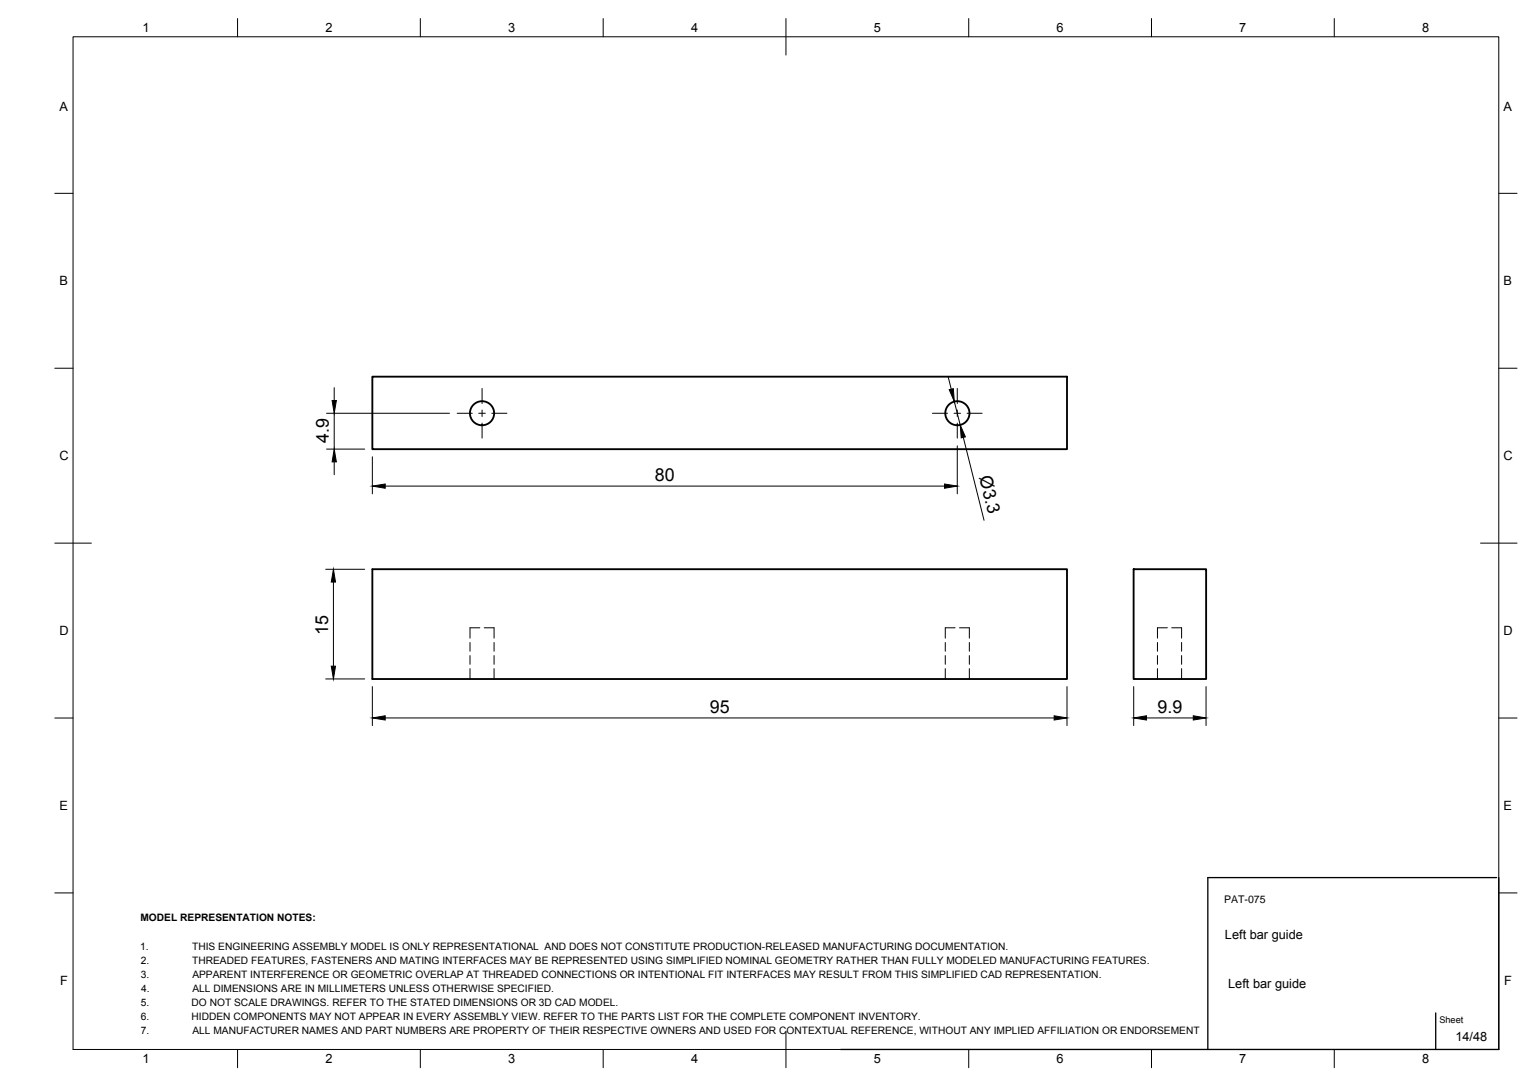
ISO-10303-21;
HEADER;
/* Generated by software containing ST-Developer
 * from STEP Tools, Inc. (www.steptools.com) 
 */

FILE_DESCRIPTION(
/* description */ ('Over-Centre Plunger Toggle Clamp on Slotted Fixture Frame'),
/* implementation_level */ '2;1');

FILE_NAME(
/* name */ 
'Left bar guide.step',
/* time_stamp */ '2026-10-28T03:23:24-07:00',
/* author */ (''),
/* organization */ (''),
/* preprocessor_version */ 'ST-DEVELOPER v20.2',
/* originating_system */ 'Autodesk Translation Framework v15.17.0.0',
/* authorisation */ '');

FILE_SCHEMA (('AUTOMOTIVE_DESIGN { 1 0 10303 214 3 1 1 }'));
ENDSEC;

DATA;
#10=MECHANICAL_DESIGN_GEOMETRIC_PRESENTATION_REPRESENTATION('',(#522),#15212);
#438=SHAPE_REPRESENTATION_RELATIONSHIP('SRR','None',#15412,#480);
#480=ADVANCED_BREP_SHAPE_REPRESENTATION('',(#573),#15174);
#522=STYLED_ITEM('',(#15712),#573);
#573=MANIFOLD_SOLID_BREP('Body1',#8254);
#708=FACE_BOUND('',#1802,.T.);
#709=FACE_BOUND('',#1803,.T.);
#846=PLANE('',#9018);
#847=PLANE('',#9022);
#848=PLANE('',#9023);
#849=PLANE('',#9024);
#850=PLANE('',#9025);
#851=PLANE('',#9026);
#852=PLANE('',#9027);
#853=PLANE('',#9028);
#1209=FACE_OUTER_BOUND('',#1792,.T.);
#1210=FACE_OUTER_BOUND('',#1793,.T.);
#1211=FACE_OUTER_BOUND('',#1794,.T.);
#1212=FACE_OUTER_BOUND('',#1795,.T.);
#1213=FACE_OUTER_BOUND('',#1796,.T.);
#1214=FACE_OUTER_BOUND('',#1797,.T.);
#1215=FACE_OUTER_BOUND('',#1798,.T.);
#1216=FACE_OUTER_BOUND('',#1799,.T.);
#1217=FACE_OUTER_BOUND('',#1800,.T.);
#1218=FACE_OUTER_BOUND('',#1801,.T.);
#1792=EDGE_LOOP('',(#6115,#6116,#6117,#6118));
#1793=EDGE_LOOP('',(#6119));
#1794=EDGE_LOOP('',(#6120,#6121,#6122,#6123));
#1795=EDGE_LOOP('',(#6124));
#1796=EDGE_LOOP('',(#6125,#6126,#6127,#6128));
#1797=EDGE_LOOP('',(#6129,#6130,#6131,#6132));
#1798=EDGE_LOOP('',(#6133,#6134,#6135,#6136));
#1799=EDGE_LOOP('',(#6137,#6138,#6139,#6140));
#1800=EDGE_LOOP('',(#6141,#6142,#6143,#6144));
#1801=EDGE_LOOP('',(#6145,#6146,#6147,#6148));
#1802=EDGE_LOOP('',(#6149));
#1803=EDGE_LOOP('',(#6150));
#2386=LINE('',#12959,#3016);
#2387=LINE('',#12966,#3017);
#2388=LINE('',#12972,#3018);
#2389=LINE('',#12974,#3019);
#2390=LINE('',#12976,#3020);
#2391=LINE('',#12977,#3021);
#2392=LINE('',#12980,#3022);
#2393=LINE('',#12982,#3023);
#2394=LINE('',#12983,#3024);
#2395=LINE('',#12986,#3025);
#2396=LINE('',#12988,#3026);
#2397=LINE('',#12989,#3027);
#2398=LINE('',#12991,#3028);
#2399=LINE('',#12992,#3029);
#3016=VECTOR('',#10417,0.165);
#3017=VECTOR('',#10426,0.165);
#3018=VECTOR('',#10433,1.);
#3019=VECTOR('',#10434,1.);
#3020=VECTOR('',#10435,1.);
#3021=VECTOR('',#10436,1.);
#3022=VECTOR('',#10439,1.);
#3023=VECTOR('',#10440,1.);
#3024=VECTOR('',#10441,1.);
#3025=VECTOR('',#10444,1.);
#3026=VECTOR('',#10445,1.);
#3027=VECTOR('',#10446,1.);
#3028=VECTOR('',#10449,1.);
#3029=VECTOR('',#10450,1.);
#3609=CIRCLE('',#9016,0.165);
#3610=CIRCLE('',#9017,0.165);
#3611=CIRCLE('',#9020,0.165);
#3612=CIRCLE('',#9021,0.165);
#4041=VERTEX_POINT('',#12956);
#4042=VERTEX_POINT('',#12958);
#4043=VERTEX_POINT('',#12963);
#4044=VERTEX_POINT('',#12965);
#4045=VERTEX_POINT('',#12970);
#4046=VERTEX_POINT('',#12971);
#4047=VERTEX_POINT('',#12973);
#4048=VERTEX_POINT('',#12975);
#4049=VERTEX_POINT('',#12979);
#4050=VERTEX_POINT('',#12981);
#4051=VERTEX_POINT('',#12985);
#4052=VERTEX_POINT('',#12987);
#4818=EDGE_CURVE('',#4041,#4041,#3609,.T.);
#4819=EDGE_CURVE('',#4041,#4042,#2386,.T.);
#4820=EDGE_CURVE('',#4042,#4042,#3610,.T.);
#4821=EDGE_CURVE('',#4043,#4043,#3611,.T.);
#4822=EDGE_CURVE('',#4043,#4044,#2387,.T.);
#4823=EDGE_CURVE('',#4044,#4044,#3612,.T.);
#4824=EDGE_CURVE('',#4045,#4046,#2388,.T.);
#4825=EDGE_CURVE('',#4046,#4047,#2389,.T.);
#4826=EDGE_CURVE('',#4048,#4047,#2390,.T.);
#4827=EDGE_CURVE('',#4045,#4048,#2391,.T.);
#4828=EDGE_CURVE('',#4049,#4045,#2392,.T.);
#4829=EDGE_CURVE('',#4050,#4048,#2393,.T.);
#4830=EDGE_CURVE('',#4049,#4050,#2394,.T.);
#4831=EDGE_CURVE('',#4051,#4049,#2395,.T.);
#4832=EDGE_CURVE('',#4052,#4050,#2396,.T.);
#4833=EDGE_CURVE('',#4051,#4052,#2397,.T.);
#4834=EDGE_CURVE('',#4046,#4051,#2398,.T.);
#4835=EDGE_CURVE('',#4047,#4052,#2399,.T.);
#6115=ORIENTED_EDGE('',*,*,#4818,.F.);
#6116=ORIENTED_EDGE('',*,*,#4819,.T.);
#6117=ORIENTED_EDGE('',*,*,#4820,.T.);
#6118=ORIENTED_EDGE('',*,*,#4819,.F.);
#6119=ORIENTED_EDGE('',*,*,#4820,.F.);
#6120=ORIENTED_EDGE('',*,*,#4821,.F.);
#6121=ORIENTED_EDGE('',*,*,#4822,.T.);
#6122=ORIENTED_EDGE('',*,*,#4823,.T.);
#6123=ORIENTED_EDGE('',*,*,#4822,.F.);
#6124=ORIENTED_EDGE('',*,*,#4823,.F.);
#6125=ORIENTED_EDGE('',*,*,#4824,.T.);
#6126=ORIENTED_EDGE('',*,*,#4825,.T.);
#6127=ORIENTED_EDGE('',*,*,#4826,.F.);
#6128=ORIENTED_EDGE('',*,*,#4827,.F.);
#6129=ORIENTED_EDGE('',*,*,#4828,.T.);
#6130=ORIENTED_EDGE('',*,*,#4827,.T.);
#6131=ORIENTED_EDGE('',*,*,#4829,.F.);
#6132=ORIENTED_EDGE('',*,*,#4830,.F.);
#6133=ORIENTED_EDGE('',*,*,#4831,.T.);
#6134=ORIENTED_EDGE('',*,*,#4830,.T.);
#6135=ORIENTED_EDGE('',*,*,#4832,.F.);
#6136=ORIENTED_EDGE('',*,*,#4833,.F.);
#6137=ORIENTED_EDGE('',*,*,#4834,.T.);
#6138=ORIENTED_EDGE('',*,*,#4833,.T.);
#6139=ORIENTED_EDGE('',*,*,#4835,.F.);
#6140=ORIENTED_EDGE('',*,*,#4825,.F.);
#6141=ORIENTED_EDGE('',*,*,#4835,.T.);
#6142=ORIENTED_EDGE('',*,*,#4832,.T.);
#6143=ORIENTED_EDGE('',*,*,#4829,.T.);
#6144=ORIENTED_EDGE('',*,*,#4826,.T.);
#6145=ORIENTED_EDGE('',*,*,#4834,.F.);
#6146=ORIENTED_EDGE('',*,*,#4824,.F.);
#6147=ORIENTED_EDGE('',*,*,#4828,.F.);
#6148=ORIENTED_EDGE('',*,*,#4831,.F.);
#6149=ORIENTED_EDGE('',*,*,#4818,.T.);
#6150=ORIENTED_EDGE('',*,*,#4821,.T.);
#7676=CYLINDRICAL_SURFACE('',#9015,0.165);
#7677=CYLINDRICAL_SURFACE('',#9019,0.165);
#7881=ADVANCED_FACE('',(#1209),#7676,.F.);
#7882=ADVANCED_FACE('',(#1210),#846,.F.);
#7883=ADVANCED_FACE('',(#1211),#7677,.F.);
#7884=ADVANCED_FACE('',(#1212),#847,.F.);
#7885=ADVANCED_FACE('',(#1213),#848,.T.);
#7886=ADVANCED_FACE('',(#1214),#849,.T.);
#7887=ADVANCED_FACE('',(#1215),#850,.T.);
#7888=ADVANCED_FACE('',(#1216),#851,.T.);
#7889=ADVANCED_FACE('',(#1217),#852,.T.);
#7890=ADVANCED_FACE('',(#1218,#708,#709),#853,.F.);
#8254=CLOSED_SHELL('',(#7881,#7882,#7883,#7884,#7885,#7886,#7887,#7888,
#7889,#7890));
#9014=AXIS2_PLACEMENT_3D('',#12954,#10411,#10412);
#9015=AXIS2_PLACEMENT_3D('',#12955,#10413,#10414);
#9016=AXIS2_PLACEMENT_3D('',#12957,#10415,#10416);
#9017=AXIS2_PLACEMENT_3D('',#12960,#10418,#10419);
#9018=AXIS2_PLACEMENT_3D('',#12961,#10420,#10421);
#9019=AXIS2_PLACEMENT_3D('',#12962,#10422,#10423);
#9020=AXIS2_PLACEMENT_3D('',#12964,#10424,#10425);
#9021=AXIS2_PLACEMENT_3D('',#12967,#10427,#10428);
#9022=AXIS2_PLACEMENT_3D('',#12968,#10429,#10430);
#9023=AXIS2_PLACEMENT_3D('',#12969,#10431,#10432);
#9024=AXIS2_PLACEMENT_3D('',#12978,#10437,#10438);
#9025=AXIS2_PLACEMENT_3D('',#12984,#10442,#10443);
#9026=AXIS2_PLACEMENT_3D('',#12990,#10447,#10448);
#9027=AXIS2_PLACEMENT_3D('',#12993,#10451,#10452);
#9028=AXIS2_PLACEMENT_3D('',#12994,#10453,#10454);
#10411=DIRECTION('axis',(0.,0.,1.));
#10412=DIRECTION('refdir',(1.,0.,0.));
#10413=DIRECTION('center_axis',(0.,0.,1.));
#10414=DIRECTION('ref_axis',(1.,0.,0.));
#10415=DIRECTION('center_axis',(0.,0.,1.));
#10416=DIRECTION('ref_axis',(1.,0.,0.));
#10417=DIRECTION('',(0.,0.,1.));
#10418=DIRECTION('center_axis',(0.,0.,1.));
#10419=DIRECTION('ref_axis',(1.,0.,0.));
#10420=DIRECTION('center_axis',(0.,0.,1.));
#10421=DIRECTION('ref_axis',(1.,0.,0.));
#10422=DIRECTION('center_axis',(0.,0.,1.));
#10423=DIRECTION('ref_axis',(1.,0.,0.));
#10424=DIRECTION('center_axis',(0.,0.,1.));
#10425=DIRECTION('ref_axis',(1.,0.,0.));
#10426=DIRECTION('',(0.,0.,1.));
#10427=DIRECTION('center_axis',(0.,0.,1.));
#10428=DIRECTION('ref_axis',(1.,0.,0.));
#10429=DIRECTION('center_axis',(0.,0.,1.));
#10430=DIRECTION('ref_axis',(1.,0.,0.));
#10431=DIRECTION('center_axis',(0.,1.,0.));
#10432=DIRECTION('ref_axis',(-1.,0.,0.));
#10433=DIRECTION('',(-1.,0.,0.));
#10434=DIRECTION('',(0.,0.,1.));
#10435=DIRECTION('',(-1.,0.,0.));
#10436=DIRECTION('',(0.,0.,1.));
#10437=DIRECTION('center_axis',(1.,0.,0.));
#10438=DIRECTION('ref_axis',(0.,1.,0.));
#10439=DIRECTION('',(0.,1.,0.));
#10440=DIRECTION('',(0.,1.,0.));
#10441=DIRECTION('',(0.,0.,1.));
#10442=DIRECTION('center_axis',(0.,-1.,0.));
#10443=DIRECTION('ref_axis',(1.,0.,0.));
#10444=DIRECTION('',(1.,0.,0.));
#10445=DIRECTION('',(1.,0.,0.));
#10446=DIRECTION('',(0.,0.,1.));
#10447=DIRECTION('center_axis',(-1.,0.,0.));
#10448=DIRECTION('ref_axis',(0.,-1.,0.));
#10449=DIRECTION('',(0.,-1.,0.));
#10450=DIRECTION('',(0.,-1.,0.));
#10451=DIRECTION('center_axis',(0.,0.,1.));
#10452=DIRECTION('ref_axis',(1.,0.,0.));
#10453=DIRECTION('center_axis',(0.,0.,1.));
#10454=DIRECTION('ref_axis',(1.,0.,0.));
#12954=CARTESIAN_POINT('',(0.,0.,0.));
#12955=CARTESIAN_POINT('Origin',(-1.5,-4.5,0.9));
#12956=CARTESIAN_POINT('',(-1.665,-4.5,1.));
#12957=CARTESIAN_POINT('Origin',(-1.5,-4.5,1.));
#12958=CARTESIAN_POINT('',(-1.665,-4.5,1.7));
#12959=CARTESIAN_POINT('',(-1.665,-4.5,0.9));
#12960=CARTESIAN_POINT('Origin',(-1.5,-4.5,1.7));
#12961=CARTESIAN_POINT('Origin',(-1.5,-4.5,1.7));
#12962=CARTESIAN_POINT('Origin',(-1.5,2.,0.9));
#12963=CARTESIAN_POINT('',(-1.665,2.,1.));
#12964=CARTESIAN_POINT('Origin',(-1.5,2.,1.));
#12965=CARTESIAN_POINT('',(-1.665,2.,1.7));
#12966=CARTESIAN_POINT('',(-1.665,2.,0.9));
#12967=CARTESIAN_POINT('Origin',(-1.5,2.,1.7));
#12968=CARTESIAN_POINT('Origin',(-1.5,2.,1.7));
#12969=CARTESIAN_POINT('Origin',(-1.01,3.5,1.));
#12970=CARTESIAN_POINT('',(-1.01,3.5,1.));
#12971=CARTESIAN_POINT('',(-2.,3.5,1.));
#12972=CARTESIAN_POINT('',(-1.01,3.5,1.));
#12973=CARTESIAN_POINT('',(-2.,3.5,2.5));
#12974=CARTESIAN_POINT('',(-2.,3.5,1.));
#12975=CARTESIAN_POINT('',(-1.01,3.5,2.5));
#12976=CARTESIAN_POINT('',(-1.01,3.5,2.5));
#12977=CARTESIAN_POINT('',(-1.01,3.5,1.));
#12978=CARTESIAN_POINT('Origin',(-1.01,-6.,1.));
#12979=CARTESIAN_POINT('',(-1.01,-6.,1.));
#12980=CARTESIAN_POINT('',(-1.01,-6.,1.));
#12981=CARTESIAN_POINT('',(-1.01,-6.,2.5));
#12982=CARTESIAN_POINT('',(-1.01,-6.,2.5));
#12983=CARTESIAN_POINT('',(-1.01,-6.,1.));
#12984=CARTESIAN_POINT('Origin',(-2.,-6.,1.));
#12985=CARTESIAN_POINT('',(-2.,-6.,1.));
#12986=CARTESIAN_POINT('',(-2.,-6.,1.));
#12987=CARTESIAN_POINT('',(-2.,-6.,2.5));
#12988=CARTESIAN_POINT('',(-2.,-6.,2.5));
#12989=CARTESIAN_POINT('',(-2.,-6.,1.));
#12990=CARTESIAN_POINT('Origin',(-2.,3.5,1.));
#12991=CARTESIAN_POINT('',(-2.,3.5,1.));
#12992=CARTESIAN_POINT('',(-2.,3.5,2.5));
#12993=CARTESIAN_POINT('Origin',(-1.505,-1.25,2.5));
#12994=CARTESIAN_POINT('Origin',(-1.505,-1.25,1.));
#15124=UNCERTAINTY_MEASURE_WITH_UNIT(LENGTH_MEASURE(0.001),#15213,
'DISTANCE_ACCURACY_VALUE',
'Maximum model space distance between geometric entities at asserted c
onnectivities');
#15162=UNCERTAINTY_MEASURE_WITH_UNIT(LENGTH_MEASURE(0.001),#15213,
'DISTANCE_ACCURACY_VALUE',
'Maximum model space distance between geometric entities at asserted c
onnectivities');
#15174=(
GEOMETRIC_REPRESENTATION_CONTEXT(3)
GLOBAL_UNCERTAINTY_ASSIGNED_CONTEXT((#15124))
GLOBAL_UNIT_ASSIGNED_CONTEXT((#15213,#15215,#15216))
REPRESENTATION_CONTEXT('','3D')
);
#15212=(
GEOMETRIC_REPRESENTATION_CONTEXT(3)
GLOBAL_UNCERTAINTY_ASSIGNED_CONTEXT((#15162))
GLOBAL_UNIT_ASSIGNED_CONTEXT((#15213,#15215,#15216))
REPRESENTATION_CONTEXT('','3D')
);
#15213=(
LENGTH_UNIT()
NAMED_UNIT(*)
SI_UNIT(.CENTI.,.METRE.)
);
#15215=(
NAMED_UNIT(*)
PLANE_ANGLE_UNIT()
SI_UNIT($,.RADIAN.)
);
#15216=(
NAMED_UNIT(*)
SI_UNIT($,.STERADIAN.)
SOLID_ANGLE_UNIT()
);
#15228=SHAPE_DEFINITION_REPRESENTATION(#15277,#15412);
#15277=PRODUCT_DEFINITION_SHAPE('',$,#15462);
#15412=SHAPE_REPRESENTATION('',(#9014),#15174);
#15450=PRODUCT_DEFINITION_CONTEXT('part definition',#15599,'design');
#15462=PRODUCT_DEFINITION('Left bar guide','Left bar guide',#15511,#15450);
#15511=PRODUCT_DEFINITION_FORMATION('',$,#15612);
#15599=APPLICATION_CONTEXT(
'Core Data for Automotive Mechanical Design Process');
#15600=PRODUCT_CONTEXT('part definition',#15599,'mechanical');
#15612=PRODUCT('Left bar guide','Left bar guide','Left bar guide',(#15600));
#15706=COLOUR_RGB('Sky Blue',0.24,0.69,0.87);
#15707=FILL_AREA_STYLE_COLOUR('',#15706);
#15708=FILL_AREA_STYLE('',(#15707));
#15709=SURFACE_STYLE_FILL_AREA(#15708);
#15710=SURFACE_SIDE_STYLE('',(#15709));
#15711=SURFACE_STYLE_USAGE(.BOTH.,#15710);
#15712=PRESENTATION_STYLE_ASSIGNMENT((#15711));
ENDSEC;
END-ISO-10303-21;
